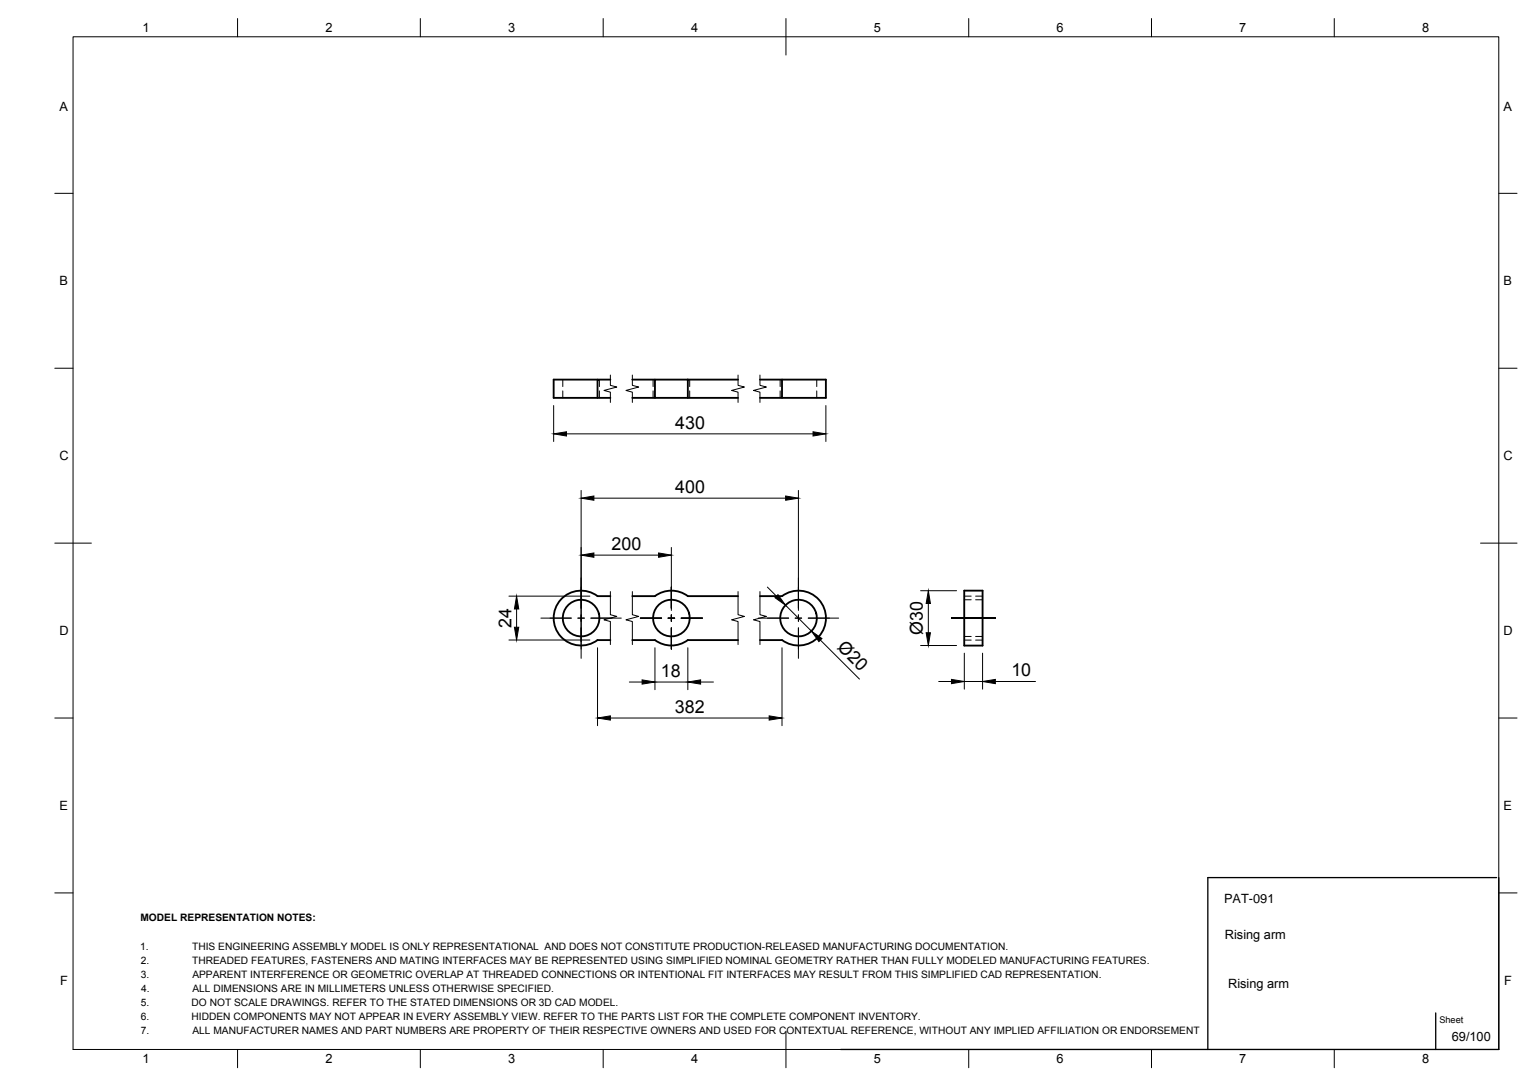
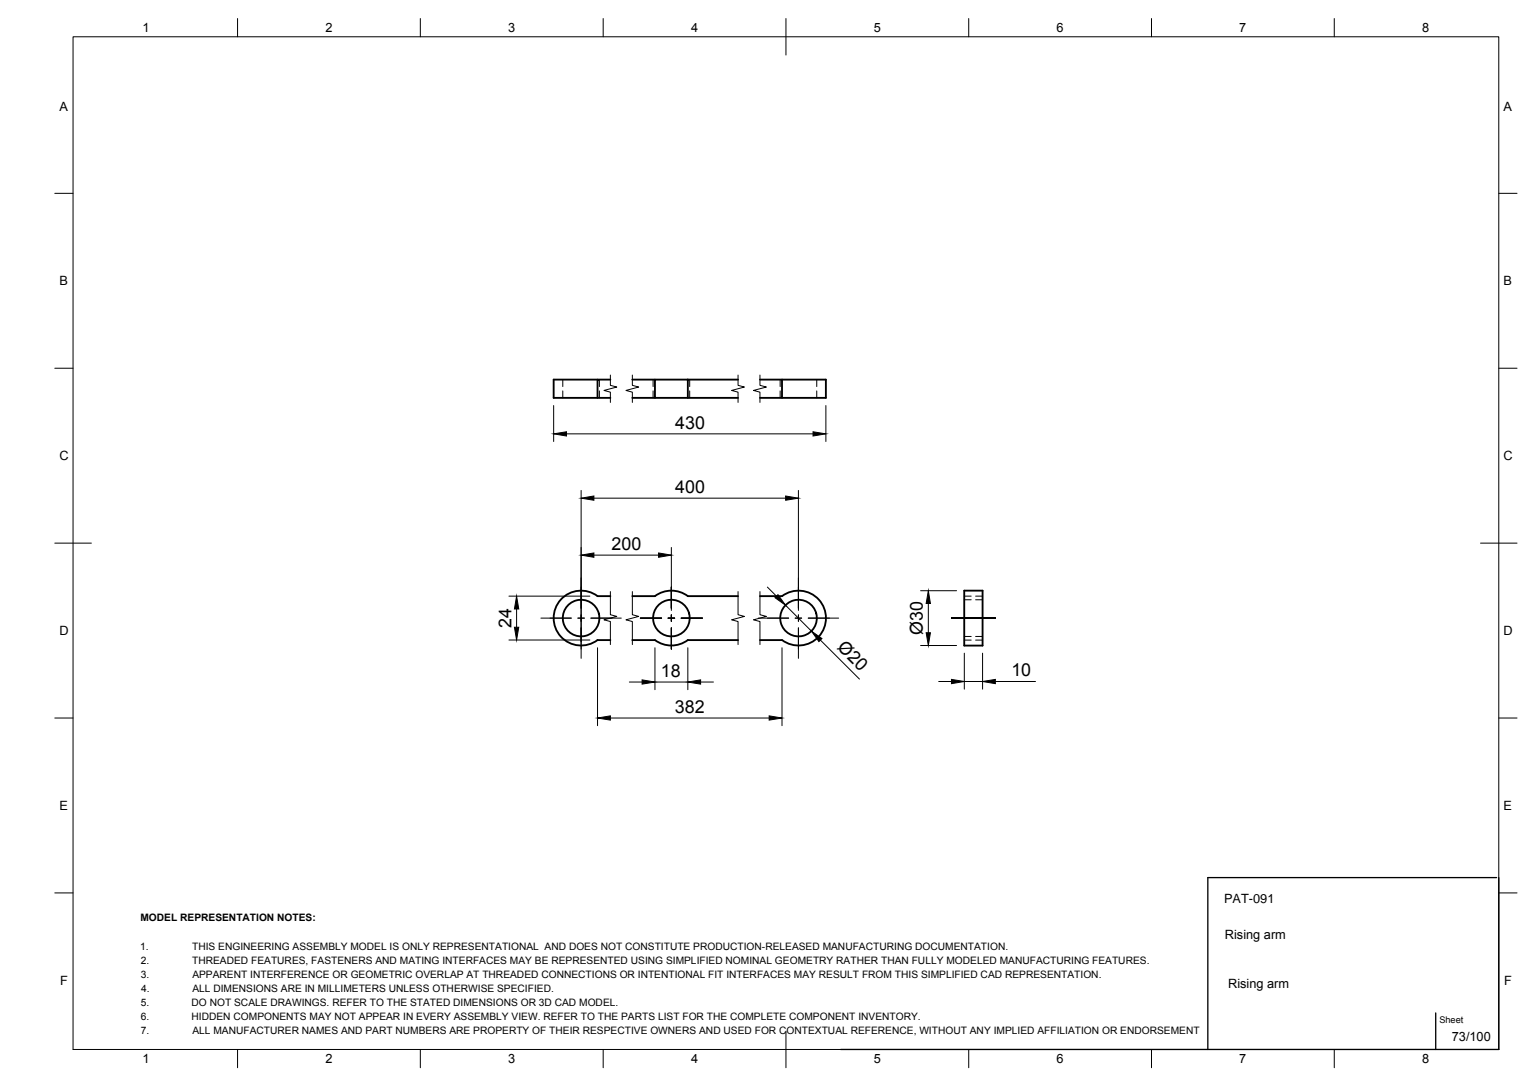
ISO-10303-21;
HEADER;
/* Generated by software containing ST-Developer
 * from STEP Tools, Inc. (www.steptools.com) 
 */

FILE_DESCRIPTION(
/* description */ ('PAT-091'),
/* implementation_level */ '2;1');

FILE_NAME(
/* name */ 'Rising arm.step',
/* time_stamp */ '2026-10-27T15:34:44-07:00',
/* author */ (''),
/* organization */ (''),
/* preprocessor_version */ 'ST-DEVELOPER v20.2',
/* originating_system */ 'Autodesk Translation Framework v15.17.0.0',
/* authorisation */ '');

FILE_SCHEMA (('AUTOMOTIVE_DESIGN { 1 0 10303 214 3 1 1 }'));
ENDSEC;

DATA;
#10=MECHANICAL_DESIGN_GEOMETRIC_PRESENTATION_REPRESENTATION('',(#1027),#25100);
#807=SHAPE_REPRESENTATION_RELATIONSHIP('SRR','None',#25573,#917);
#917=ADVANCED_BREP_SHAPE_REPRESENTATION('',(#1149),#25043);
#1027=STYLED_ITEM('',(#26177),#1149);
#1149=MANIFOLD_SOLID_BREP('Body1',#13306);
#1484=FACE_BOUND('',#3607,.T.);
#1485=FACE_BOUND('',#3608,.T.);
#1486=FACE_BOUND('',#3609,.T.);
#1487=FACE_BOUND('',#3614,.T.);
#1488=FACE_BOUND('',#3615,.T.);
#1489=FACE_BOUND('',#3616,.T.);
#1895=PLANE('',#15496);
#1896=PLANE('',#15497);
#1897=PLANE('',#15498);
#1898=PLANE('',#15505);
#1899=PLANE('',#15508);
#1900=PLANE('',#15513);
#2511=FACE_OUTER_BOUND('',#3598,.T.);
#2512=FACE_OUTER_BOUND('',#3599,.T.);
#2513=FACE_OUTER_BOUND('',#3600,.T.);
#2514=FACE_OUTER_BOUND('',#3601,.T.);
#2515=FACE_OUTER_BOUND('',#3602,.T.);
#2516=FACE_OUTER_BOUND('',#3603,.T.);
#2517=FACE_OUTER_BOUND('',#3604,.T.);
#2518=FACE_OUTER_BOUND('',#3605,.T.);
#2519=FACE_OUTER_BOUND('',#3606,.T.);
#2520=FACE_OUTER_BOUND('',#3610,.T.);
#2521=FACE_OUTER_BOUND('',#3611,.T.);
#2522=FACE_OUTER_BOUND('',#3612,.T.);
#2523=FACE_OUTER_BOUND('',#3613,.T.);
#3598=EDGE_LOOP('',(#10774,#10775,#10776,#10777));
#3599=EDGE_LOOP('',(#10778,#10779,#10780,#10781));
#3600=EDGE_LOOP('',(#10782,#10783,#10784,#10785));
#3601=EDGE_LOOP('',(#10786,#10787,#10788,#10789));
#3602=EDGE_LOOP('',(#10790,#10791,#10792,#10793));
#3603=EDGE_LOOP('',(#10794,#10795,#10796,#10797));
#3604=EDGE_LOOP('',(#10798,#10799,#10800,#10801));
#3605=EDGE_LOOP('',(#10802,#10803,#10804,#10805));
#3606=EDGE_LOOP('',(#10806,#10807,#10808,#10809,#10810,#10811,#10812,#10813));
#3607=EDGE_LOOP('',(#10814));
#3608=EDGE_LOOP('',(#10815));
#3609=EDGE_LOOP('',(#10816));
#3610=EDGE_LOOP('',(#10817,#10818,#10819,#10820));
#3611=EDGE_LOOP('',(#10821,#10822,#10823,#10824));
#3612=EDGE_LOOP('',(#10825,#10826,#10827,#10828));
#3613=EDGE_LOOP('',(#10829,#10830,#10831,#10832,#10833,#10834,#10835,#10836));
#3614=EDGE_LOOP('',(#10837));
#3615=EDGE_LOOP('',(#10838));
#3616=EDGE_LOOP('',(#10839));
#4633=LINE('',#23043,#5373);
#4634=LINE('',#23048,#5374);
#4635=LINE('',#23052,#5375);
#4636=LINE('',#23057,#5376);
#4637=LINE('',#23061,#5377);
#4638=LINE('',#23065,#5378);
#4639=LINE('',#23067,#5379);
#4640=LINE('',#23068,#5380);
#4641=LINE('',#23071,#5381);
#4642=LINE('',#23073,#5382);
#4643=LINE('',#23074,#5383);
#4644=LINE('',#23077,#5384);
#4645=LINE('',#23079,#5385);
#4646=LINE('',#23080,#5386);
#4647=LINE('',#23085,#5387);
#4648=LINE('',#23092,#5388);
#4649=LINE('',#23098,#5389);
#4650=LINE('',#23099,#5390);
#4651=LINE('',#23102,#5391);
#5373=VECTOR('',#18785,1.);
#5374=VECTOR('',#18790,1.);
#5375=VECTOR('',#18793,1.);
#5376=VECTOR('',#18798,1.);
#5377=VECTOR('',#18801,1.);
#5378=VECTOR('',#18806,1.);
#5379=VECTOR('',#18807,1.);
#5380=VECTOR('',#18808,1.);
#5381=VECTOR('',#18811,1.);
#5382=VECTOR('',#18812,1.);
#5383=VECTOR('',#18813,1.);
#5384=VECTOR('',#18816,1.);
#5385=VECTOR('',#18817,1.);
#5386=VECTOR('',#18818,1.);
#5387=VECTOR('',#18823,1.);
#5388=VECTOR('',#18834,1.);
#5389=VECTOR('',#18841,1.);
#5390=VECTOR('',#18842,1.);
#5391=VECTOR('',#18845,1.);
#5992=CIRCLE('',#15488,1.);
#5993=CIRCLE('',#15489,1.);
#5994=CIRCLE('',#15491,1.5);
#5995=CIRCLE('',#15492,1.5);
#5996=CIRCLE('',#15494,1.5);
#5997=CIRCLE('',#15495,1.5);
#5998=CIRCLE('',#15500,1.);
#5999=CIRCLE('',#15501,1.);
#6000=CIRCLE('',#15503,1.5);
#6001=CIRCLE('',#15504,1.5);
#6002=CIRCLE('',#15506,1.5);
#6003=CIRCLE('',#15507,1.);
#6004=CIRCLE('',#15510,1.);
#6005=CIRCLE('',#15512,1.5);
#6981=VERTEX_POINT('',#23040);
#6982=VERTEX_POINT('',#23042);
#6983=VERTEX_POINT('',#23046);
#6984=VERTEX_POINT('',#23047);
#6985=VERTEX_POINT('',#23049);
#6986=VERTEX_POINT('',#23051);
#6987=VERTEX_POINT('',#23055);
#6988=VERTEX_POINT('',#23056);
#6989=VERTEX_POINT('',#23058);
#6990=VERTEX_POINT('',#23060);
#6991=VERTEX_POINT('',#23064);
#6992=VERTEX_POINT('',#23066);
#6993=VERTEX_POINT('',#23070);
#6994=VERTEX_POINT('',#23072);
#6995=VERTEX_POINT('',#23076);
#6996=VERTEX_POINT('',#23078);
#6997=VERTEX_POINT('',#23082);
#6998=VERTEX_POINT('',#23084);
#6999=VERTEX_POINT('',#23091);
#7000=VERTEX_POINT('',#23094);
#7001=VERTEX_POINT('',#23097);
#7002=VERTEX_POINT('',#23101);
#8322=EDGE_CURVE('',#6981,#6981,#5992,.T.);
#8323=EDGE_CURVE('',#6981,#6982,#4633,.T.);
#8324=EDGE_CURVE('',#6982,#6982,#5993,.T.);
#8325=EDGE_CURVE('',#6983,#6984,#4634,.T.);
#8326=EDGE_CURVE('',#6983,#6985,#5994,.T.);
#8327=EDGE_CURVE('',#6986,#6985,#4635,.T.);
#8328=EDGE_CURVE('',#6984,#6986,#5995,.T.);
#8329=EDGE_CURVE('',#6987,#6988,#4636,.T.);
#8330=EDGE_CURVE('',#6989,#6987,#5996,.T.);
#8331=EDGE_CURVE('',#6990,#6989,#4637,.T.);
#8332=EDGE_CURVE('',#6990,#6988,#5997,.T.);
#8333=EDGE_CURVE('',#6991,#6989,#4638,.T.);
#8334=EDGE_CURVE('',#6991,#6992,#4639,.T.);
#8335=EDGE_CURVE('',#6992,#6990,#4640,.T.);
#8336=EDGE_CURVE('',#6988,#6993,#4641,.T.);
#8337=EDGE_CURVE('',#6993,#6994,#4642,.T.);
#8338=EDGE_CURVE('',#6987,#6994,#4643,.T.);
#8339=EDGE_CURVE('',#6985,#6995,#4644,.T.);
#8340=EDGE_CURVE('',#6995,#6996,#4645,.T.);
#8341=EDGE_CURVE('',#6986,#6996,#4646,.T.);
#8342=EDGE_CURVE('',#6997,#6997,#5998,.T.);
#8343=EDGE_CURVE('',#6997,#6998,#4647,.T.);
#8344=EDGE_CURVE('',#6998,#6998,#5999,.T.);
#8345=EDGE_CURVE('',#6996,#6991,#6000,.T.);
#8346=EDGE_CURVE('',#6995,#6992,#6001,.T.);
#8347=EDGE_CURVE('',#6999,#6983,#4648,.T.);
#8348=EDGE_CURVE('',#6993,#6999,#6002,.T.);
#8349=EDGE_CURVE('',#7000,#7000,#6003,.T.);
#8350=EDGE_CURVE('',#7001,#6984,#4649,.T.);
#8351=EDGE_CURVE('',#7001,#6999,#4650,.T.);
#8352=EDGE_CURVE('',#7000,#7002,#4651,.T.);
#8353=EDGE_CURVE('',#7002,#7002,#6004,.T.);
#8354=EDGE_CURVE('',#6994,#7001,#6005,.T.);
#10774=ORIENTED_EDGE('',*,*,#8322,.F.);
#10775=ORIENTED_EDGE('',*,*,#8323,.T.);
#10776=ORIENTED_EDGE('',*,*,#8324,.F.);
#10777=ORIENTED_EDGE('',*,*,#8323,.F.);
#10778=ORIENTED_EDGE('',*,*,#8325,.F.);
#10779=ORIENTED_EDGE('',*,*,#8326,.T.);
#10780=ORIENTED_EDGE('',*,*,#8327,.F.);
#10781=ORIENTED_EDGE('',*,*,#8328,.F.);
#10782=ORIENTED_EDGE('',*,*,#8329,.F.);
#10783=ORIENTED_EDGE('',*,*,#8330,.F.);
#10784=ORIENTED_EDGE('',*,*,#8331,.F.);
#10785=ORIENTED_EDGE('',*,*,#8332,.T.);
#10786=ORIENTED_EDGE('',*,*,#8331,.T.);
#10787=ORIENTED_EDGE('',*,*,#8333,.F.);
#10788=ORIENTED_EDGE('',*,*,#8334,.T.);
#10789=ORIENTED_EDGE('',*,*,#8335,.T.);
#10790=ORIENTED_EDGE('',*,*,#8329,.T.);
#10791=ORIENTED_EDGE('',*,*,#8336,.T.);
#10792=ORIENTED_EDGE('',*,*,#8337,.T.);
#10793=ORIENTED_EDGE('',*,*,#8338,.F.);
#10794=ORIENTED_EDGE('',*,*,#8327,.T.);
#10795=ORIENTED_EDGE('',*,*,#8339,.T.);
#10796=ORIENTED_EDGE('',*,*,#8340,.T.);
#10797=ORIENTED_EDGE('',*,*,#8341,.F.);
#10798=ORIENTED_EDGE('',*,*,#8342,.F.);
#10799=ORIENTED_EDGE('',*,*,#8343,.T.);
#10800=ORIENTED_EDGE('',*,*,#8344,.F.);
#10801=ORIENTED_EDGE('',*,*,#8343,.F.);
#10802=ORIENTED_EDGE('',*,*,#8334,.F.);
#10803=ORIENTED_EDGE('',*,*,#8345,.F.);
#10804=ORIENTED_EDGE('',*,*,#8340,.F.);
#10805=ORIENTED_EDGE('',*,*,#8346,.T.);
#10806=ORIENTED_EDGE('',*,*,#8347,.F.);
#10807=ORIENTED_EDGE('',*,*,#8348,.F.);
#10808=ORIENTED_EDGE('',*,*,#8336,.F.);
#10809=ORIENTED_EDGE('',*,*,#8332,.F.);
#10810=ORIENTED_EDGE('',*,*,#8335,.F.);
#10811=ORIENTED_EDGE('',*,*,#8346,.F.);
#10812=ORIENTED_EDGE('',*,*,#8339,.F.);
#10813=ORIENTED_EDGE('',*,*,#8326,.F.);
#10814=ORIENTED_EDGE('',*,*,#8322,.T.);
#10815=ORIENTED_EDGE('',*,*,#8342,.T.);
#10816=ORIENTED_EDGE('',*,*,#8349,.T.);
#10817=ORIENTED_EDGE('',*,*,#8325,.T.);
#10818=ORIENTED_EDGE('',*,*,#8350,.F.);
#10819=ORIENTED_EDGE('',*,*,#8351,.T.);
#10820=ORIENTED_EDGE('',*,*,#8347,.T.);
#10821=ORIENTED_EDGE('',*,*,#8349,.F.);
#10822=ORIENTED_EDGE('',*,*,#8352,.T.);
#10823=ORIENTED_EDGE('',*,*,#8353,.F.);
#10824=ORIENTED_EDGE('',*,*,#8352,.F.);
#10825=ORIENTED_EDGE('',*,*,#8337,.F.);
#10826=ORIENTED_EDGE('',*,*,#8348,.T.);
#10827=ORIENTED_EDGE('',*,*,#8351,.F.);
#10828=ORIENTED_EDGE('',*,*,#8354,.F.);
#10829=ORIENTED_EDGE('',*,*,#8338,.T.);
#10830=ORIENTED_EDGE('',*,*,#8354,.T.);
#10831=ORIENTED_EDGE('',*,*,#8350,.T.);
#10832=ORIENTED_EDGE('',*,*,#8328,.T.);
#10833=ORIENTED_EDGE('',*,*,#8341,.T.);
#10834=ORIENTED_EDGE('',*,*,#8345,.T.);
#10835=ORIENTED_EDGE('',*,*,#8333,.T.);
#10836=ORIENTED_EDGE('',*,*,#8330,.T.);
#10837=ORIENTED_EDGE('',*,*,#8324,.T.);
#10838=ORIENTED_EDGE('',*,*,#8344,.T.);
#10839=ORIENTED_EDGE('',*,*,#8353,.T.);
#12259=CYLINDRICAL_SURFACE('',#15487,1.);
#12260=CYLINDRICAL_SURFACE('',#15490,1.5);
#12261=CYLINDRICAL_SURFACE('',#15493,1.5);
#12262=CYLINDRICAL_SURFACE('',#15499,1.);
#12263=CYLINDRICAL_SURFACE('',#15502,1.5);
#12264=CYLINDRICAL_SURFACE('',#15509,1.);
#12265=CYLINDRICAL_SURFACE('',#15511,1.5);
#12878=ADVANCED_FACE('',(#2511),#12259,.F.);
#12879=ADVANCED_FACE('',(#2512),#12260,.T.);
#12880=ADVANCED_FACE('',(#2513),#12261,.T.);
#12881=ADVANCED_FACE('',(#2514),#1895,.T.);
#12882=ADVANCED_FACE('',(#2515),#1896,.T.);
#12883=ADVANCED_FACE('',(#2516),#1897,.T.);
#12884=ADVANCED_FACE('',(#2517),#12262,.F.);
#12885=ADVANCED_FACE('',(#2518),#12263,.T.);
#12886=ADVANCED_FACE('',(#2519,#1484,#1485,#1486),#1898,.F.);
#12887=ADVANCED_FACE('',(#2520),#1899,.T.);
#12888=ADVANCED_FACE('',(#2521),#12264,.F.);
#12889=ADVANCED_FACE('',(#2522),#12265,.T.);
#12890=ADVANCED_FACE('',(#2523,#1487,#1488,#1489),#1900,.T.);
#13306=CLOSED_SHELL('',(#12878,#12879,#12880,#12881,#12882,#12883,#12884,
#12885,#12886,#12887,#12888,#12889,#12890));
#15486=AXIS2_PLACEMENT_3D('',#23038,#18779,#18780);
#15487=AXIS2_PLACEMENT_3D('',#23039,#18781,#18782);
#15488=AXIS2_PLACEMENT_3D('',#23041,#18783,#18784);
#15489=AXIS2_PLACEMENT_3D('',#23044,#18786,#18787);
#15490=AXIS2_PLACEMENT_3D('',#23045,#18788,#18789);
#15491=AXIS2_PLACEMENT_3D('',#23050,#18791,#18792);
#15492=AXIS2_PLACEMENT_3D('',#23053,#18794,#18795);
#15493=AXIS2_PLACEMENT_3D('',#23054,#18796,#18797);
#15494=AXIS2_PLACEMENT_3D('',#23059,#18799,#18800);
#15495=AXIS2_PLACEMENT_3D('',#23062,#18802,#18803);
#15496=AXIS2_PLACEMENT_3D('',#23063,#18804,#18805);
#15497=AXIS2_PLACEMENT_3D('',#23069,#18809,#18810);
#15498=AXIS2_PLACEMENT_3D('',#23075,#18814,#18815);
#15499=AXIS2_PLACEMENT_3D('',#23081,#18819,#18820);
#15500=AXIS2_PLACEMENT_3D('',#23083,#18821,#18822);
#15501=AXIS2_PLACEMENT_3D('',#23086,#18824,#18825);
#15502=AXIS2_PLACEMENT_3D('',#23087,#18826,#18827);
#15503=AXIS2_PLACEMENT_3D('',#23088,#18828,#18829);
#15504=AXIS2_PLACEMENT_3D('',#23089,#18830,#18831);
#15505=AXIS2_PLACEMENT_3D('',#23090,#18832,#18833);
#15506=AXIS2_PLACEMENT_3D('',#23093,#18835,#18836);
#15507=AXIS2_PLACEMENT_3D('',#23095,#18837,#18838);
#15508=AXIS2_PLACEMENT_3D('',#23096,#18839,#18840);
#15509=AXIS2_PLACEMENT_3D('',#23100,#18843,#18844);
#15510=AXIS2_PLACEMENT_3D('',#23103,#18846,#18847);
#15511=AXIS2_PLACEMENT_3D('',#23104,#18848,#18849);
#15512=AXIS2_PLACEMENT_3D('',#23105,#18850,#18851);
#15513=AXIS2_PLACEMENT_3D('',#23106,#18852,#18853);
#18779=DIRECTION('axis',(0.,0.,1.));
#18780=DIRECTION('refdir',(1.,0.,0.));
#18781=DIRECTION('center_axis',(0.,1.,0.));
#18782=DIRECTION('ref_axis',(1.,0.,0.));
#18783=DIRECTION('center_axis',(0.,1.,0.));
#18784=DIRECTION('ref_axis',(1.,0.,0.));
#18785=DIRECTION('',(0.,1.,0.));
#18786=DIRECTION('center_axis',(0.,-1.,0.));
#18787=DIRECTION('ref_axis',(1.,0.,0.));
#18788=DIRECTION('center_axis',(0.,1.,0.));
#18789=DIRECTION('ref_axis',(1.,0.,0.));
#18790=DIRECTION('',(0.,1.,0.));
#18791=DIRECTION('center_axis',(0.,1.,0.));
#18792=DIRECTION('ref_axis',(1.,0.,0.));
#18793=DIRECTION('',(0.,-1.,0.));
#18794=DIRECTION('center_axis',(0.,1.,0.));
#18795=DIRECTION('ref_axis',(1.,0.,0.));
#18796=DIRECTION('center_axis',(0.,1.,0.));
#18797=DIRECTION('ref_axis',(1.,0.,0.));
#18798=DIRECTION('',(0.,-1.,0.));
#18799=DIRECTION('center_axis',(0.,1.,0.));
#18800=DIRECTION('ref_axis',(1.,0.,0.));
#18801=DIRECTION('',(0.,1.,0.));
#18802=DIRECTION('center_axis',(0.,1.,0.));
#18803=DIRECTION('ref_axis',(1.,0.,0.));
#18804=DIRECTION('center_axis',(0.25,0.,-0.968245836551854));
#18805=DIRECTION('ref_axis',(-0.968245836551854,0.,-0.25));
#18806=DIRECTION('',(-0.968245836551854,0.,-0.25));
#18807=DIRECTION('',(0.,-1.,0.));
#18808=DIRECTION('',(-0.968245836551854,0.,-0.25));
#18809=DIRECTION('center_axis',(0.25,0.,-0.968245836551854));
#18810=DIRECTION('ref_axis',(-0.968245836551854,0.,-0.25));
#18811=DIRECTION('',(-0.968245836551854,0.,-0.25));
#18812=DIRECTION('',(0.,1.,0.));
#18813=DIRECTION('',(-0.968245836551854,0.,-0.25));
#18814=DIRECTION('center_axis',(-0.25,0.,0.968245836551854));
#18815=DIRECTION('ref_axis',(0.968245836551854,0.,0.25));
#18816=DIRECTION('',(0.968245836551854,0.,0.25));
#18817=DIRECTION('',(0.,1.,0.));
#18818=DIRECTION('',(0.968245836551854,0.,0.25));
#18819=DIRECTION('center_axis',(0.,1.,0.));
#18820=DIRECTION('ref_axis',(1.,0.,0.));
#18821=DIRECTION('center_axis',(0.,1.,0.));
#18822=DIRECTION('ref_axis',(1.,0.,0.));
#18823=DIRECTION('',(0.,1.,0.));
#18824=DIRECTION('center_axis',(0.,-1.,0.));
#18825=DIRECTION('ref_axis',(1.,0.,0.));
#18826=DIRECTION('center_axis',(0.,1.,0.));
#18827=DIRECTION('ref_axis',(1.,0.,0.));
#18828=DIRECTION('center_axis',(0.,1.,0.));
#18829=DIRECTION('ref_axis',(1.,0.,0.));
#18830=DIRECTION('center_axis',(0.,1.,0.));
#18831=DIRECTION('ref_axis',(1.,0.,0.));
#18832=DIRECTION('center_axis',(0.,1.,0.));
#18833=DIRECTION('ref_axis',(1.,0.,0.));
#18834=DIRECTION('',(0.968245836551854,0.,0.25));
#18835=DIRECTION('center_axis',(0.,1.,0.));
#18836=DIRECTION('ref_axis',(1.,0.,0.));
#18837=DIRECTION('center_axis',(0.,1.,0.));
#18838=DIRECTION('ref_axis',(1.,0.,0.));
#18839=DIRECTION('center_axis',(-0.25,0.,0.968245836551854));
#18840=DIRECTION('ref_axis',(0.968245836551854,0.,0.25));
#18841=DIRECTION('',(0.968245836551854,0.,0.25));
#18842=DIRECTION('',(0.,-1.,0.));
#18843=DIRECTION('center_axis',(0.,1.,0.));
#18844=DIRECTION('ref_axis',(1.,0.,0.));
#18845=DIRECTION('',(0.,1.,0.));
#18846=DIRECTION('center_axis',(0.,-1.,0.));
#18847=DIRECTION('ref_axis',(1.,0.,0.));
#18848=DIRECTION('center_axis',(0.,1.,0.));
#18849=DIRECTION('ref_axis',(-0.968245836551854,0.,-0.250000000000002));
#18850=DIRECTION('center_axis',(0.,1.,0.));
#18851=DIRECTION('ref_axis',(1.,0.,0.));
#18852=DIRECTION('center_axis',(0.,1.,0.));
#18853=DIRECTION('ref_axis',(0.,0.,1.));
#23038=CARTESIAN_POINT('',(0.,0.,0.));
#23039=CARTESIAN_POINT('Origin',(19.3649167310371,-7.1,8.));
#23040=CARTESIAN_POINT('',(18.3649167310371,-7.,8.));
#23041=CARTESIAN_POINT('Origin',(19.3649167310371,-7.,8.));
#23042=CARTESIAN_POINT('',(18.3649167310371,-6.,8.));
#23043=CARTESIAN_POINT('',(18.3649167310371,-7.1,8.));
#23044=CARTESIAN_POINT('Origin',(19.3649167310371,-6.,8.));
#23045=CARTESIAN_POINT('Origin',(19.3649167310371,-7.,8.));
#23046=CARTESIAN_POINT('',(18.1934954781404,-7.,8.93689500386222));
#23047=CARTESIAN_POINT('',(18.1934954781404,-6.,8.93689500386223));
#23048=CARTESIAN_POINT('',(18.1934954781404,-7.,8.93689500386223));
#23049=CARTESIAN_POINT('',(19.9363379839338,-7.,9.38689500386222));
#23050=CARTESIAN_POINT('Origin',(19.3649167310371,-7.,8.));
#23051=CARTESIAN_POINT('',(19.9363379839338,-6.,9.38689500386223));
#23052=CARTESIAN_POINT('',(19.9363379839338,-7.,9.38689500386223));
#23053=CARTESIAN_POINT('Origin',(19.3649167310371,-6.,8.));
#23054=CARTESIAN_POINT('Origin',(19.3649167310371,-7.,8.));
#23055=CARTESIAN_POINT('',(18.7934954781404,-6.,6.61310499613778));
#23056=CARTESIAN_POINT('',(18.7934954781404,-7.,6.61310499613778));
#23057=CARTESIAN_POINT('',(18.7934954781404,-7.,6.61310499613778));
#23058=CARTESIAN_POINT('',(20.5363379839338,-6.,7.06310499613778));
#23059=CARTESIAN_POINT('Origin',(19.3649167310371,-6.,8.));
#23060=CARTESIAN_POINT('',(20.5363379839338,-7.,7.06310499613778));
#23061=CARTESIAN_POINT('',(20.5363379839338,-7.,7.06310499613778));
#23062=CARTESIAN_POINT('Origin',(19.3649167310371,-7.,8.));
#23063=CARTESIAN_POINT('Origin',(39.0298334620742,-7.,11.8381049961378));
#23064=CARTESIAN_POINT('',(38.1584122091775,-6.,11.6131049961378));
#23065=CARTESIAN_POINT('',(39.0298334620742,-6.,11.8381049961378));
#23066=CARTESIAN_POINT('',(38.1584122091775,-7.,11.6131049961378));
#23067=CARTESIAN_POINT('',(38.1584122091775,-7.,11.6131049961378));
#23068=CARTESIAN_POINT('',(39.0298334620742,-7.,11.8381049961378));
#23069=CARTESIAN_POINT('Origin',(39.0298334620742,-7.,11.8381049961378));
#23070=CARTESIAN_POINT('',(1.17142125289667,-7.,2.06310499613778));
#23071=CARTESIAN_POINT('',(39.0298334620742,-7.,11.8381049961378));
#23072=CARTESIAN_POINT('',(1.17142125289667,-6.,2.06310499613778));
#23073=CARTESIAN_POINT('',(1.17142125289667,-7.,2.06310499613778));
#23074=CARTESIAN_POINT('',(39.0298334620742,-6.,11.8381049961378));
#23075=CARTESIAN_POINT('Origin',(-0.3,-7.,4.16189500386223));
#23076=CARTESIAN_POINT('',(37.5584122091775,-7.,13.9368950038622));
#23077=CARTESIAN_POINT('',(-0.3,-7.,4.16189500386223));
#23078=CARTESIAN_POINT('',(37.5584122091775,-6.,13.9368950038622));
#23079=CARTESIAN_POINT('',(37.5584122091775,-7.,13.9368950038622));
#23080=CARTESIAN_POINT('',(-0.3,-6.,4.16189500386223));
#23081=CARTESIAN_POINT('Origin',(38.7298334620742,-7.1,13.));
#23082=CARTESIAN_POINT('',(37.7298334620742,-7.,13.));
#23083=CARTESIAN_POINT('Origin',(38.7298334620742,-7.,13.));
#23084=CARTESIAN_POINT('',(37.7298334620742,-6.,13.));
#23085=CARTESIAN_POINT('',(37.7298334620742,-7.1,13.));
#23086=CARTESIAN_POINT('Origin',(38.7298334620742,-6.,13.));
#23087=CARTESIAN_POINT('Origin',(38.7298334620742,-7.,13.));
#23088=CARTESIAN_POINT('Origin',(38.7298334620742,-6.,13.));
#23089=CARTESIAN_POINT('Origin',(38.7298334620742,-7.,13.));
#23090=CARTESIAN_POINT('Origin',(19.3649167310371,-7.,8.));
#23091=CARTESIAN_POINT('',(0.571421252896668,-7.,4.38689500386223));
#23092=CARTESIAN_POINT('',(-0.3,-7.,4.16189500386223));
#23093=CARTESIAN_POINT('Origin',(0.,-7.,3.));
#23094=CARTESIAN_POINT('',(-1.,-7.,3.));
#23095=CARTESIAN_POINT('Origin',(0.,-7.,3.));
#23096=CARTESIAN_POINT('Origin',(-0.3,-7.,4.16189500386223));
#23097=CARTESIAN_POINT('',(0.571421252896668,-6.,4.38689500386223));
#23098=CARTESIAN_POINT('',(-0.3,-6.,4.16189500386223));
#23099=CARTESIAN_POINT('',(0.571421252896668,-7.,4.38689500386223));
#23100=CARTESIAN_POINT('Origin',(0.,-7.1,3.));
#23101=CARTESIAN_POINT('',(-1.,-6.,3.));
#23102=CARTESIAN_POINT('',(-1.,-7.1,3.));
#23103=CARTESIAN_POINT('Origin',(0.,-6.,3.));
#23104=CARTESIAN_POINT('Origin',(0.,-7.,3.));
#23105=CARTESIAN_POINT('Origin',(0.,-6.,3.));
#23106=CARTESIAN_POINT('Origin',(19.3649167310371,-6.,8.));
#24922=UNCERTAINTY_MEASURE_WITH_UNIT(LENGTH_MEASURE(0.001),#25101,
'DISTANCE_ACCURACY_VALUE',
'Maximum model space distance between geometric entities at asserted c
onnectivities');
#24979=UNCERTAINTY_MEASURE_WITH_UNIT(LENGTH_MEASURE(0.001),#25101,
'DISTANCE_ACCURACY_VALUE',
'Maximum model space distance between geometric entities at asserted c
onnectivities');
#25043=(
GEOMETRIC_REPRESENTATION_CONTEXT(3)
GLOBAL_UNCERTAINTY_ASSIGNED_CONTEXT((#24922))
GLOBAL_UNIT_ASSIGNED_CONTEXT((#25101,#25103,#25104))
REPRESENTATION_CONTEXT('','3D')
);
#25100=(
GEOMETRIC_REPRESENTATION_CONTEXT(3)
GLOBAL_UNCERTAINTY_ASSIGNED_CONTEXT((#24979))
GLOBAL_UNIT_ASSIGNED_CONTEXT((#25101,#25103,#25104))
REPRESENTATION_CONTEXT('','3D')
);
#25101=(
LENGTH_UNIT()
NAMED_UNIT(*)
SI_UNIT(.CENTI.,.METRE.)
);
#25103=(
NAMED_UNIT(*)
PLANE_ANGLE_UNIT()
SI_UNIT($,.RADIAN.)
);
#25104=(
NAMED_UNIT(*)
SI_UNIT($,.STERADIAN.)
SOLID_ANGLE_UNIT()
);
#25168=SHAPE_DEFINITION_REPRESENTATION(#25290,#25573);
#25290=PRODUCT_DEFINITION_SHAPE('',$,#25694);
#25573=SHAPE_REPRESENTATION('',(#15486),#25043);
#25630=PRODUCT_DEFINITION_CONTEXT('part definition',#25992,'design');
#25694=PRODUCT_DEFINITION('Rising arm','Rising arm',#25814,#25630);
#25814=PRODUCT_DEFINITION_FORMATION('',$,#26057);
#25992=APPLICATION_CONTEXT(
'Core Data for Automotive Mechanical Design Process');
#25993=PRODUCT_CONTEXT('part definition',#25992,'mechanical');
#26057=PRODUCT('Rising arm','Rising arm','Rising arm',(#25993));
#26171=COLOUR_RGB('Light Blue',0.38,0.62,0.78);
#26172=FILL_AREA_STYLE_COLOUR('',#26171);
#26173=FILL_AREA_STYLE('',(#26172));
#26174=SURFACE_STYLE_FILL_AREA(#26173);
#26175=SURFACE_SIDE_STYLE('',(#26174));
#26176=SURFACE_STYLE_USAGE(.BOTH.,#26175);
#26177=PRESENTATION_STYLE_ASSIGNMENT((#26176));
ENDSEC;
END-ISO-10303-21;
